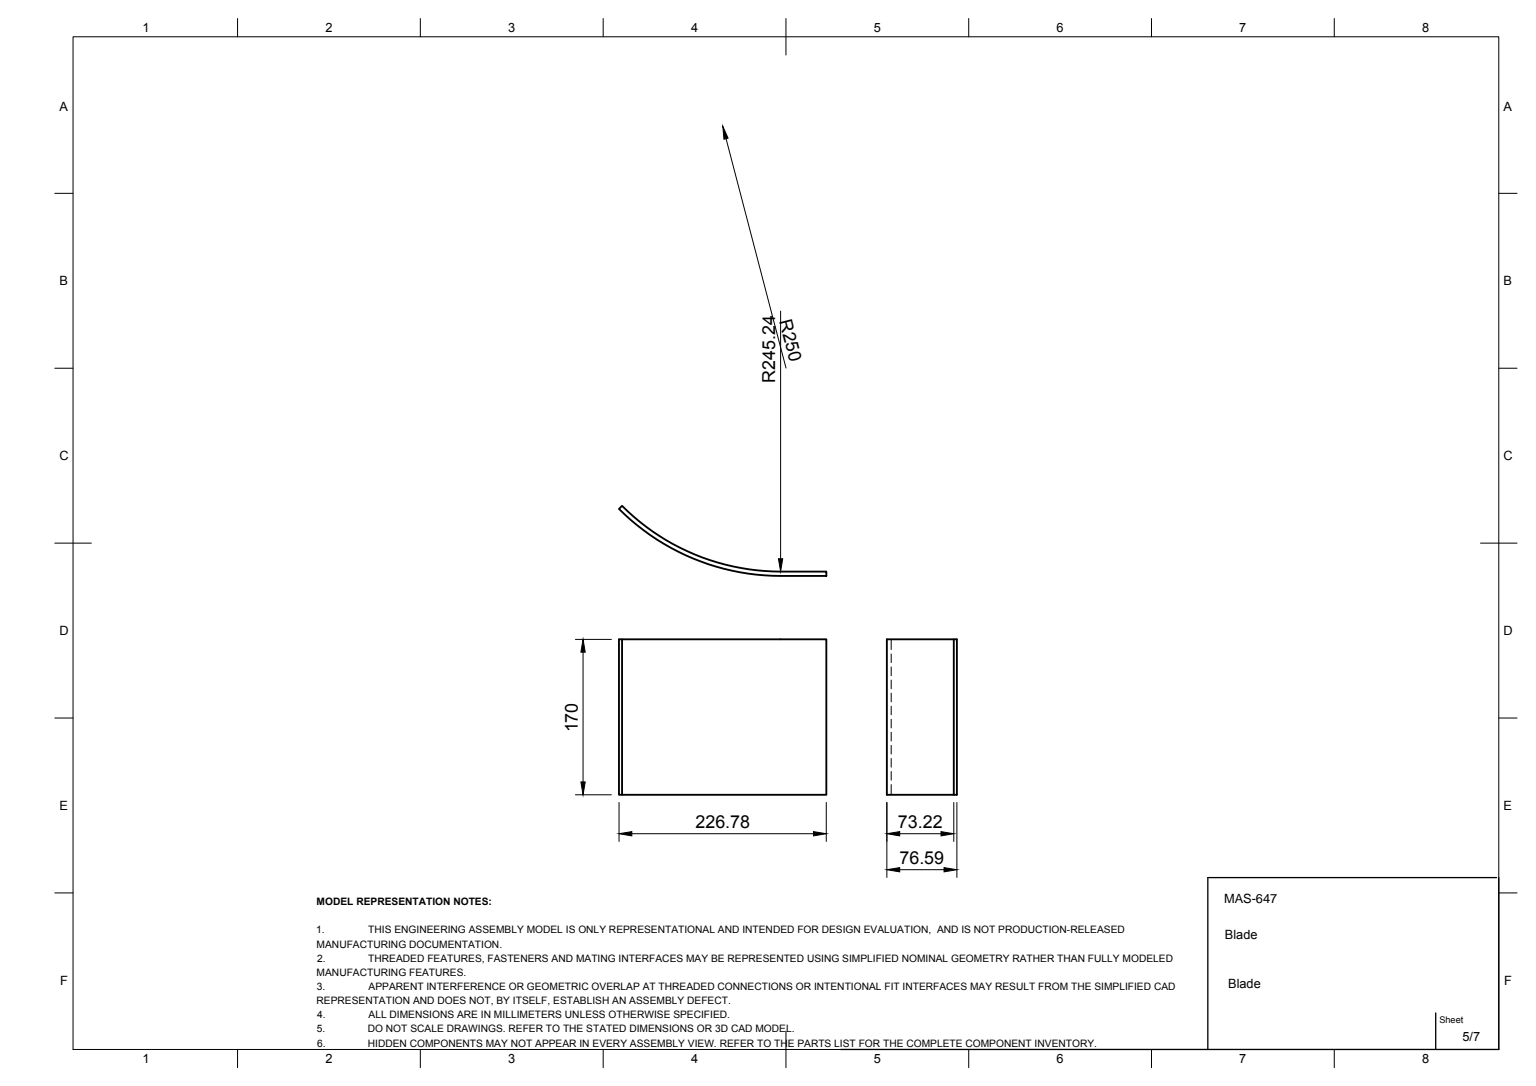
ISO-10303-21;
HEADER;
FILE_DESCRIPTION((''),'2;1');
FILE_NAME('Blade.step','2026-10-09T11:36:02-07:00',(''),(''),'','','');
FILE_SCHEMA (('AUTOMOTIVE_DESIGN { 1 0 10303 214 3 1 1 }'));
ENDSEC;
DATA;
#10=MECHANICAL_DESIGN_GEOMETRIC_PRESENTATION_REPRESENTATION('',(#86),#1549);
#76=SHAPE_REPRESENTATION_RELATIONSHIP('SRR','None',#1585,#81) ;
#81=ADVANCED_BREP_SHAPE_REPRESENTATION('',(#91),#1548) ;
#86=STYLED_ITEM('',(#1615),#91) ;
#91=MANIFOLD_SOLID_BREP('Body1',#848) ;
#133=PLANE('',#995) ;
#134=PLANE('',#998) ;
#135=PLANE('',#1001) ;
#136=PLANE('',#1002) ;
#137=PLANE('',#1003) ;
#138=PLANE('',#1005) ;
#139=PLANE('',#1007) ;
#140=PLANE('',#1008) ;
#177=FACE_OUTER_BOUND('',#254,.T.) ;
#178=FACE_OUTER_BOUND('',#255,.T.) ;
#179=FACE_OUTER_BOUND('',#256,.T.) ;
#180=FACE_OUTER_BOUND('',#257,.T.) ;
#181=FACE_OUTER_BOUND('',#258,.T.) ;
#182=FACE_OUTER_BOUND('',#259,.T.) ;
#183=FACE_OUTER_BOUND('',#260,.T.) ;
#184=FACE_OUTER_BOUND('',#261,.T.) ;
#185=FACE_OUTER_BOUND('',#262,.T.) ;
#186=FACE_OUTER_BOUND('',#263,.T.) ;
#254=EDGE_LOOP('',(#735,#736,#737,#738)) ;
#255=EDGE_LOOP('',(#739,#740,#741,#742)) ;
#256=EDGE_LOOP('',(#743,#744,#745,#746)) ;
#257=EDGE_LOOP('',(#747,#748,#749,#750)) ;
#258=EDGE_LOOP('',(#751,#752,#753,#754)) ;
#259=EDGE_LOOP('',(#755,#756,#757,#758)) ;
#260=EDGE_LOOP('',(#759,#760,#761,#762)) ;
#261=EDGE_LOOP('',(#763,#764,#765,#766)) ;
#262=EDGE_LOOP('',(#767,#768,#769,#770)) ;
#263=EDGE_LOOP('',(#771,#772,#773,#774)) ;
#296=LINE('',#1483,#344) ;
#297=LINE('',#1487,#345) ;
#298=LINE('',#1492,#346) ;
#299=LINE('',#1496,#347) ;
#300=LINE('',#1500,#348) ;
#301=LINE('',#1502,#349) ;
#302=LINE('',#1503,#350) ;
#303=LINE('',#1504,#351) ;
#304=LINE('',#1507,#352) ;
#305=LINE('',#1509,#353) ;
#306=LINE('',#1510,#354) ;
#307=LINE('',#1512,#355) ;
#308=LINE('',#1513,#356) ;
#309=LINE('',#1514,#357) ;
#310=LINE('',#1516,#358) ;
#311=LINE('',#1518,#359) ;
#344=VECTOR('',#1237,1000.) ;
#345=VECTOR('',#1240,1000.) ;
#346=VECTOR('',#1245,1000.) ;
#347=VECTOR('',#1248,1000.) ;
#348=VECTOR('',#1253,1000.) ;
#349=VECTOR('',#1254,1000.) ;
#350=VECTOR('',#1255,1000.) ;
#351=VECTOR('',#1256,1000.) ;
#352=VECTOR('',#1259,1000.) ;
#353=VECTOR('',#1260,1000.) ;
#354=VECTOR('',#1261,1000.) ;
#355=VECTOR('',#1264,1000.) ;
#356=VECTOR('',#1265,1000.) ;
#357=VECTOR('',#1266,1000.) ;
#358=VECTOR('',#1269,1000.) ;
#359=VECTOR('',#1272,1000.) ;
#408=CIRCLE('',#996,250.) ;
#409=CIRCLE('',#997,245.24) ;
#410=CIRCLE('',#999,245.24) ;
#411=CIRCLE('',#1000,250.) ;
#463=VERTEX_POINT('',#1481) ;
#464=VERTEX_POINT('',#1482) ;
#465=VERTEX_POINT('',#1484) ;
#466=VERTEX_POINT('',#1486) ;
#467=VERTEX_POINT('',#1490) ;
#468=VERTEX_POINT('',#1491) ;
#469=VERTEX_POINT('',#1493) ;
#470=VERTEX_POINT('',#1495) ;
#471=VERTEX_POINT('',#1499) ;
#472=VERTEX_POINT('',#1501) ;
#473=VERTEX_POINT('',#1506) ;
#474=VERTEX_POINT('',#1508) ;
#555=EDGE_CURVE('',#463,#464,#296,.T.) ;
#556=EDGE_CURVE('',#465,#463,#408,.T.) ;
#557=EDGE_CURVE('',#466,#465,#297,.T.) ;
#558=EDGE_CURVE('',#466,#464,#409,.T.) ;
#559=EDGE_CURVE('',#467,#468,#298,.T.) ;
#560=EDGE_CURVE('',#469,#467,#410,.T.) ;
#561=EDGE_CURVE('',#469,#470,#299,.T.) ;
#562=EDGE_CURVE('',#470,#468,#411,.T.) ;
#563=EDGE_CURVE('',#467,#471,#300,.T.) ;
#564=EDGE_CURVE('',#472,#471,#301,.T.) ;
#565=EDGE_CURVE('',#464,#472,#302,.T.) ;
#566=EDGE_CURVE('',#464,#467,#303,.T.) ;
#567=EDGE_CURVE('',#473,#471,#304,.T.) ;
#568=EDGE_CURVE('',#474,#473,#305,.T.) ;
#569=EDGE_CURVE('',#474,#472,#306,.T.) ;
#570=EDGE_CURVE('',#468,#473,#307,.T.) ;
#571=EDGE_CURVE('',#463,#468,#308,.T.) ;
#572=EDGE_CURVE('',#463,#474,#309,.T.) ;
#573=EDGE_CURVE('',#465,#470,#310,.T.) ;
#574=EDGE_CURVE('',#466,#469,#311,.T.) ;
#735=ORIENTED_EDGE('',*,*,#555,.F.) ;
#736=ORIENTED_EDGE('',*,*,#556,.F.) ;
#737=ORIENTED_EDGE('',*,*,#557,.F.) ;
#738=ORIENTED_EDGE('',*,*,#558,.T.) ;
#739=ORIENTED_EDGE('',*,*,#559,.F.) ;
#740=ORIENTED_EDGE('',*,*,#560,.F.) ;
#741=ORIENTED_EDGE('',*,*,#561,.T.) ;
#742=ORIENTED_EDGE('',*,*,#562,.T.) ;
#743=ORIENTED_EDGE('',*,*,#563,.T.) ;
#744=ORIENTED_EDGE('',*,*,#564,.F.) ;
#745=ORIENTED_EDGE('',*,*,#565,.F.) ;
#746=ORIENTED_EDGE('',*,*,#566,.T.) ;
#747=ORIENTED_EDGE('',*,*,#567,.F.) ;
#748=ORIENTED_EDGE('',*,*,#568,.F.) ;
#749=ORIENTED_EDGE('',*,*,#569,.T.) ;
#750=ORIENTED_EDGE('',*,*,#564,.T.) ;
#751=ORIENTED_EDGE('',*,*,#570,.F.) ;
#752=ORIENTED_EDGE('',*,*,#571,.F.) ;
#753=ORIENTED_EDGE('',*,*,#572,.T.) ;
#754=ORIENTED_EDGE('',*,*,#568,.T.) ;
#755=ORIENTED_EDGE('',*,*,#562,.F.) ;
#756=ORIENTED_EDGE('',*,*,#573,.F.) ;
#757=ORIENTED_EDGE('',*,*,#556,.T.) ;
#758=ORIENTED_EDGE('',*,*,#571,.T.) ;
#759=ORIENTED_EDGE('',*,*,#561,.F.) ;
#760=ORIENTED_EDGE('',*,*,#574,.F.) ;
#761=ORIENTED_EDGE('',*,*,#557,.T.) ;
#762=ORIENTED_EDGE('',*,*,#573,.T.) ;
#763=ORIENTED_EDGE('',*,*,#560,.T.) ;
#764=ORIENTED_EDGE('',*,*,#566,.F.) ;
#765=ORIENTED_EDGE('',*,*,#558,.F.) ;
#766=ORIENTED_EDGE('',*,*,#574,.T.) ;
#767=ORIENTED_EDGE('',*,*,#565,.T.) ;
#768=ORIENTED_EDGE('',*,*,#569,.F.) ;
#769=ORIENTED_EDGE('',*,*,#572,.F.) ;
#770=ORIENTED_EDGE('',*,*,#555,.T.) ;
#771=ORIENTED_EDGE('',*,*,#563,.F.) ;
#772=ORIENTED_EDGE('',*,*,#559,.T.) ;
#773=ORIENTED_EDGE('',*,*,#570,.T.) ;
#774=ORIENTED_EDGE('',*,*,#567,.T.) ;
#796=CYLINDRICAL_SURFACE('',#1004,250.) ;
#797=CYLINDRICAL_SURFACE('',#1006,245.24) ;
#834=ADVANCED_FACE('',(#177),#133,.T.) ;
#835=ADVANCED_FACE('',(#178),#134,.T.) ;
#836=ADVANCED_FACE('',(#179),#135,.F.) ;
#837=ADVANCED_FACE('',(#180),#136,.T.) ;
#838=ADVANCED_FACE('',(#181),#137,.T.) ;
#839=ADVANCED_FACE('',(#182),#796,.T.) ;
#840=ADVANCED_FACE('',(#183),#138,.T.) ;
#841=ADVANCED_FACE('',(#184),#797,.F.) ;
#842=ADVANCED_FACE('',(#185),#139,.F.) ;
#843=ADVANCED_FACE('',(#186),#140,.T.) ;
#848=CLOSED_SHELL('',(#834,#835,#836,#837,#838,#839,#840,#841,#842,#843)) ;
#994=AXIS2_PLACEMENT_3D('',#1479,#1233,#1234) ;
#995=AXIS2_PLACEMENT_3D('',#1480,#1235,#1236) ;
#996=AXIS2_PLACEMENT_3D('',#1485,#1238,#1239) ;
#997=AXIS2_PLACEMENT_3D('',#1488,#1241,#1242) ;
#998=AXIS2_PLACEMENT_3D('',#1489,#1243,#1244) ;
#999=AXIS2_PLACEMENT_3D('',#1494,#1246,#1247) ;
#1000=AXIS2_PLACEMENT_3D('',#1497,#1249,#1250) ;
#1001=AXIS2_PLACEMENT_3D('',#1498,#1251,#1252) ;
#1002=AXIS2_PLACEMENT_3D('',#1505,#1257,#1258) ;
#1003=AXIS2_PLACEMENT_3D('',#1511,#1262,#1263) ;
#1004=AXIS2_PLACEMENT_3D('',#1515,#1267,#1268) ;
#1005=AXIS2_PLACEMENT_3D('',#1517,#1270,#1271) ;
#1006=AXIS2_PLACEMENT_3D('',#1519,#1273,#1274) ;
#1007=AXIS2_PLACEMENT_3D('',#1520,#1275,#1276) ;
#1008=AXIS2_PLACEMENT_3D('',#1521,#1277,#1278) ;
#1233=DIRECTION('axis',(0.,0.,1.)) ;
#1234=DIRECTION('refdir',(1.,0.,0.)) ;
#1235=DIRECTION('center_axis',(1.,0.,0.)) ;
#1236=DIRECTION('ref_axis',(0.,0.,-1.)) ;
#1237=DIRECTION('',(0.,-1.,0.)) ;
#1238=DIRECTION('center_axis',(-1.,0.,0.)) ;
#1239=DIRECTION('ref_axis',(0.,0.,1.)) ;
#1240=DIRECTION('',(0.,0.70710678118655,0.707106781186545)) ;
#1241=DIRECTION('center_axis',(-1.,0.,0.)) ;
#1242=DIRECTION('ref_axis',(0.,1.77635683940025E-15,-1.)) ;
#1243=DIRECTION('center_axis',(-1.,0.,0.)) ;
#1244=DIRECTION('ref_axis',(0.,0.,1.)) ;
#1245=DIRECTION('',(0.,1.,0.)) ;
#1246=DIRECTION('center_axis',(-1.,0.,0.)) ;
#1247=DIRECTION('ref_axis',(0.,1.77635683940025E-15,-1.)) ;
#1248=DIRECTION('',(0.,0.70710678118655,0.707106781186545)) ;
#1249=DIRECTION('center_axis',(-1.,0.,0.)) ;
#1250=DIRECTION('ref_axis',(0.,0.,1.)) ;
#1251=DIRECTION('center_axis',(0.,1.,0.)) ;
#1252=DIRECTION('ref_axis',(0.,0.,1.)) ;
#1253=DIRECTION('',(0.,0.,-1.)) ;
#1254=DIRECTION('',(-1.,0.,0.)) ;
#1255=DIRECTION('',(0.,0.,-1.)) ;
#1256=DIRECTION('',(-1.,0.,0.)) ;
#1257=DIRECTION('center_axis',(0.,0.,-1.)) ;
#1258=DIRECTION('ref_axis',(-1.,0.,0.)) ;
#1259=DIRECTION('',(0.,-1.,0.)) ;
#1260=DIRECTION('',(-1.,0.,0.)) ;
#1261=DIRECTION('',(0.,-1.,0.)) ;
#1262=DIRECTION('center_axis',(0.,1.,0.)) ;
#1263=DIRECTION('ref_axis',(0.,0.,1.)) ;
#1264=DIRECTION('',(0.,0.,-1.)) ;
#1265=DIRECTION('',(-1.,0.,0.)) ;
#1266=DIRECTION('',(0.,0.,-1.)) ;
#1267=DIRECTION('center_axis',(-1.,0.,0.)) ;
#1268=DIRECTION('ref_axis',(0.,0.,1.)) ;
#1269=DIRECTION('',(-1.,0.,0.)) ;
#1270=DIRECTION('center_axis',(0.,-0.707106781186545,0.70710678118655)) ;
#1271=DIRECTION('ref_axis',(0.,-0.70710678118655,-0.707106781186545)) ;
#1272=DIRECTION('',(-1.,0.,0.)) ;
#1273=DIRECTION('center_axis',(-1.,0.,0.)) ;
#1274=DIRECTION('ref_axis',(0.,0.,1.)) ;
#1275=DIRECTION('center_axis',(-1.,0.,0.)) ;
#1276=DIRECTION('ref_axis',(0.,0.,1.)) ;
#1277=DIRECTION('center_axis',(-1.,0.,0.)) ;
#1278=DIRECTION('ref_axis',(0.,0.,1.)) ;
#1479=CARTESIAN_POINT('',(0.,0.,0.)) ;
#1480=CARTESIAN_POINT('Origin',(85.,250.,5.55111512312578E-14)) ;
#1481=CARTESIAN_POINT('',(85.,250.,5.55111512312578E-14)) ;
#1482=CARTESIAN_POINT('',(85.,245.240000000001,-1.11022302462516E-13)) ;
#1483=CARTESIAN_POINT('',(85.,250.,5.55111512312578E-14)) ;
#1484=CARTESIAN_POINT('',(85.,176.776695296637,176.776695296638)) ;
#1485=CARTESIAN_POINT('Origin',(85.,0.,0.)) ;
#1486=CARTESIAN_POINT('',(85.,173.410867018189,173.41086701819)) ;
#1487=CARTESIAN_POINT('',(85.,173.410867018189,173.41086701819)) ;
#1488=CARTESIAN_POINT('Origin',(85.,0.,0.)) ;
#1489=CARTESIAN_POINT('Origin',(-85.,245.240000000001,-1.11022302462516E-13)) ;
#1490=CARTESIAN_POINT('',(-85.,245.240000000001,-1.11022302462516E-13)) ;
#1491=CARTESIAN_POINT('',(-85.,250.,5.55111512312578E-14)) ;
#1492=CARTESIAN_POINT('',(-85.,245.240000000001,-1.11022302462516E-13)) ;
#1493=CARTESIAN_POINT('',(-85.,173.410867018189,173.41086701819)) ;
#1494=CARTESIAN_POINT('Origin',(-85.,0.,0.)) ;
#1495=CARTESIAN_POINT('',(-85.,176.776695296637,176.776695296638)) ;
#1496=CARTESIAN_POINT('',(-85.,173.410867018189,173.41086701819)) ;
#1497=CARTESIAN_POINT('Origin',(-85.,0.,0.)) ;
#1498=CARTESIAN_POINT('Origin',(85.,245.240000000001,-1.11022302462516E-13)) ;
#1499=CARTESIAN_POINT('',(-85.,245.24,-50.0000000000003)) ;
#1500=CARTESIAN_POINT('',(-85.,245.240000000001,-1.11022302462516E-13)) ;
#1501=CARTESIAN_POINT('',(85.,245.24,-50.0000000000003)) ;
#1502=CARTESIAN_POINT('',(85.,245.24,-50.0000000000003)) ;
#1503=CARTESIAN_POINT('',(85.,245.240000000001,-1.11022302462516E-13)) ;
#1504=CARTESIAN_POINT('',(85.,245.240000000001,-1.11022302462516E-13)) ;
#1505=CARTESIAN_POINT('Origin',(85.,250.,-50.0000000000002)) ;
#1506=CARTESIAN_POINT('',(-85.,250.,-50.0000000000002)) ;
#1507=CARTESIAN_POINT('',(-85.,250.,-50.0000000000002)) ;
#1508=CARTESIAN_POINT('',(85.,250.,-50.0000000000002)) ;
#1509=CARTESIAN_POINT('',(85.,250.,-50.0000000000002)) ;
#1510=CARTESIAN_POINT('',(85.,250.,-50.0000000000002)) ;
#1511=CARTESIAN_POINT('Origin',(85.,250.,5.55111512312578E-14)) ;
#1512=CARTESIAN_POINT('',(-85.,250.,5.55111512312578E-14)) ;
#1513=CARTESIAN_POINT('',(85.,250.,5.55111512312578E-14)) ;
#1514=CARTESIAN_POINT('',(85.,250.,5.55111512312578E-14)) ;
#1515=CARTESIAN_POINT('Origin',(85.,0.,0.)) ;
#1516=CARTESIAN_POINT('',(85.,176.776695296637,176.776695296638)) ;
#1517=CARTESIAN_POINT('Origin',(85.,173.410867018189,173.41086701819)) ;
#1518=CARTESIAN_POINT('',(85.,173.410867018189,173.41086701819)) ;
#1519=CARTESIAN_POINT('Origin',(85.,0.,0.)) ;
#1520=CARTESIAN_POINT('Origin',(85.,0.,0.)) ;
#1521=CARTESIAN_POINT('Origin',(-85.,0.,0.)) ;
#1541=UNCERTAINTY_MEASURE_WITH_UNIT(LENGTH_MEASURE(0.01),#1550,
'DISTANCE_ACCURACY_VALUE',
'Maximum model space distance between geometric entities at asserted c
onnectivities') ;
#1542=UNCERTAINTY_MEASURE_WITH_UNIT(LENGTH_MEASURE(0.01),#1550,
'DISTANCE_ACCURACY_VALUE',
'Maximum model space distance between geometric entities at asserted c
onnectivities') ;
#1548=(
GEOMETRIC_REPRESENTATION_CONTEXT(3)
GLOBAL_UNCERTAINTY_ASSIGNED_CONTEXT((#1541))
GLOBAL_UNIT_ASSIGNED_CONTEXT((#1550,#1552,#1553))
REPRESENTATION_CONTEXT('','3D')
) ;
#1549=(
GEOMETRIC_REPRESENTATION_CONTEXT(3)
GLOBAL_UNCERTAINTY_ASSIGNED_CONTEXT((#1542))
GLOBAL_UNIT_ASSIGNED_CONTEXT((#1550,#1552,#1553))
REPRESENTATION_CONTEXT('','3D')
) ;
#1550=(
LENGTH_UNIT()
NAMED_UNIT(*)
SI_UNIT(.MILLI.,.METRE.)
) ;
#1552=(
NAMED_UNIT(*)
PLANE_ANGLE_UNIT()
SI_UNIT($,.RADIAN.)
) ;
#1553=(
NAMED_UNIT(*)
SI_UNIT($,.STERADIAN.)
SOLID_ANGLE_UNIT()
) ;
#1559=SHAPE_DEFINITION_REPRESENTATION(#1565,#1585) ;
#1565=PRODUCT_DEFINITION_SHAPE('',$,#1592) ;
#1585=SHAPE_REPRESENTATION('',(#994),#1548) ;
#1586=PRODUCT_DEFINITION_CONTEXT('part definition',#1606,'design') ;
#1592=PRODUCT_DEFINITION('Blade','Blade',#1598,#1586) ;
#1598=PRODUCT_DEFINITION_FORMATION('',$,#1613) ;
#1606=APPLICATION_CONTEXT(
'Core Data for Automotive Mechanical Design Process') ;
#1607=PRODUCT_CONTEXT('part definition',#1606,'mechanical') ;
#1613=PRODUCT('Blade','Blade',$,(#1607)) ;
#1615=PRESENTATION_STYLE_ASSIGNMENT((#1617)) ;
#1617=SURFACE_STYLE_USAGE(.BOTH.,#1619) ;
#1619=SURFACE_SIDE_STYLE('',(#1621)) ;
#1621=SURFACE_STYLE_FILL_AREA(#1623) ;
#1623=FILL_AREA_STYLE('Opaque(202,209,238)',(#1625)) ;
#1625=FILL_AREA_STYLE_COLOUR('Opaque(202,209,238)',#1627) ;
#1627=COLOUR_RGB('Opaque(202,209,238)', 0.09019608, 0.27058824, 0.51372549) ;
ENDSEC;
END-ISO-10303-21;
